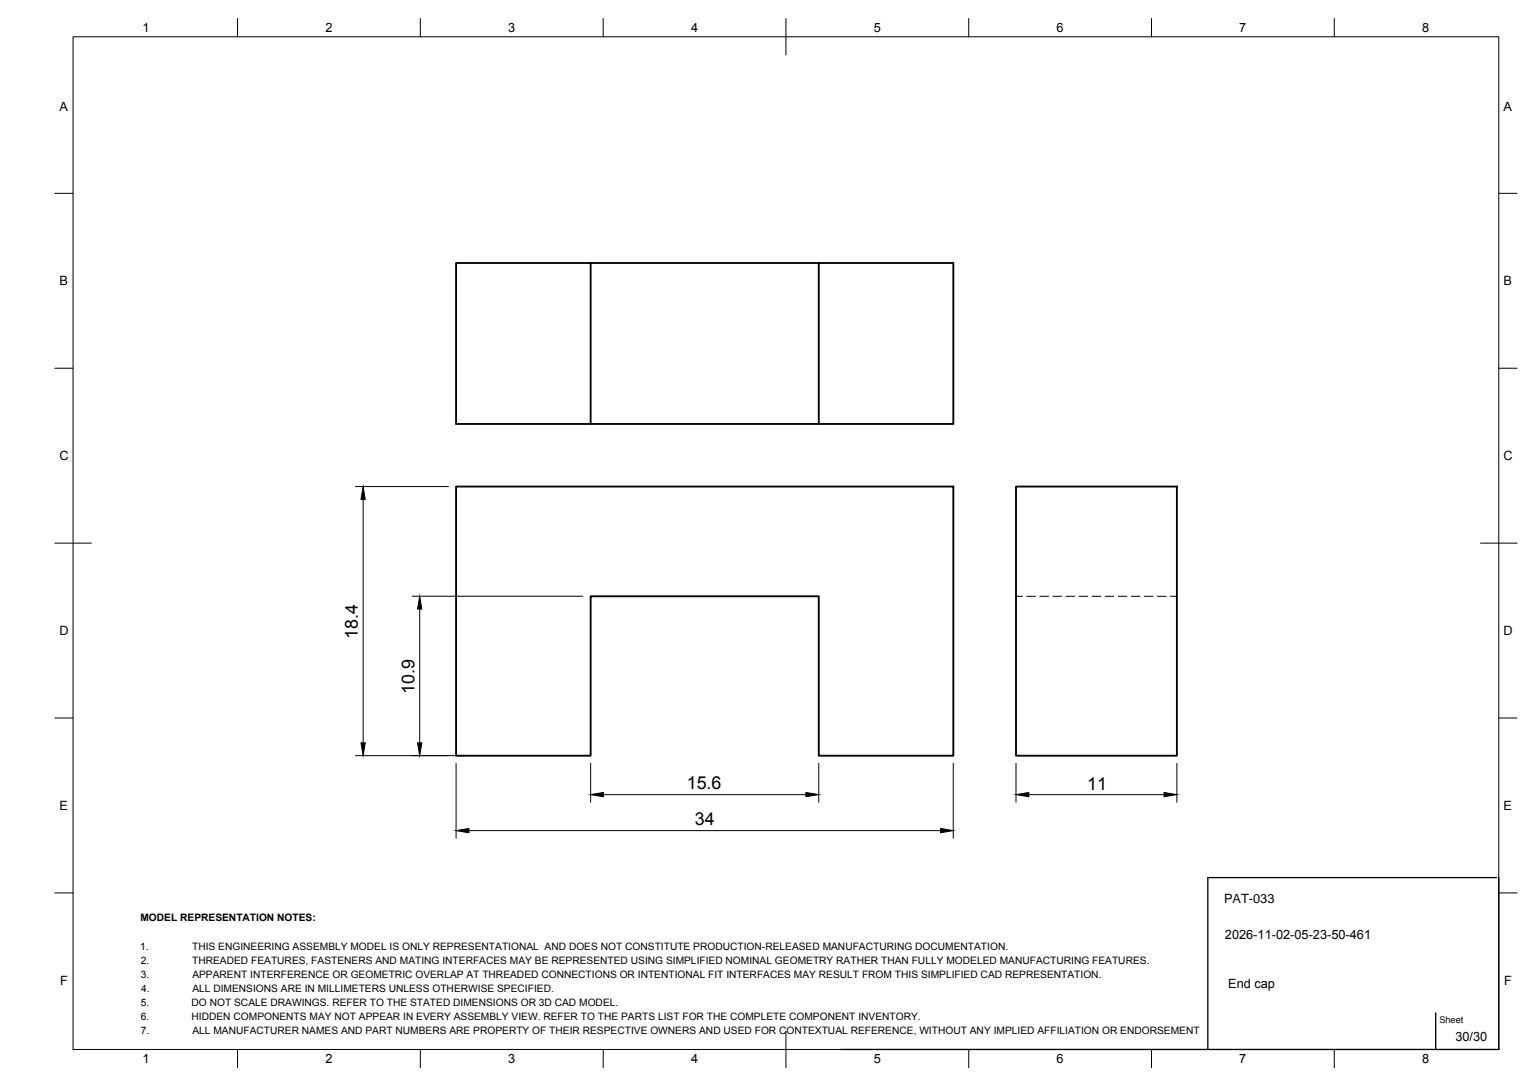
ISO-10303-21;
HEADER;
/* Generated by software containing ST-Developer
 * from STEP Tools, Inc. (www.steptools.com) 
 */

FILE_DESCRIPTION(
/* description */ ('Dual-rail gantry carriage'),
/* implementation_level */ '2;1');

FILE_NAME(
/* name */ 'End cap.step',
/* time_stamp */ '2026-10-27T10:49:15-07:00',
/* author */ (''),
/* organization */ (''),
/* preprocessor_version */ 'ST-DEVELOPER v20.2',
/* originating_system */ 'Autodesk Translation Framework v15.17.0.0',
/* authorisation */ '');

FILE_SCHEMA (('AUTOMOTIVE_DESIGN { 1 0 10303 214 3 1 1 }'));
ENDSEC;

DATA;
#10=MECHANICAL_DESIGN_GEOMETRIC_PRESENTATION_REPRESENTATION('',(#609),#12804);
#547=SHAPE_REPRESENTATION_RELATIONSHIP('SRR','None',#13027,#578);
#578=ADVANCED_BREP_SHAPE_REPRESENTATION('',(#638),#12797);
#609=STYLED_ITEM('',(#13261),#638);
#638=MANIFOLD_SOLID_BREP('Body1',#7389);
#999=PLANE('',#8250);
#1000=PLANE('',#8251);
#1001=PLANE('',#8252);
#1002=PLANE('',#8253);
#1003=PLANE('',#8254);
#1004=PLANE('',#8255);
#1005=PLANE('',#8256);
#1006=PLANE('',#8257);
#1007=PLANE('',#8258);
#1008=PLANE('',#8259);
#1363=FACE_OUTER_BOUND('',#1865,.T.);
#1364=FACE_OUTER_BOUND('',#1866,.T.);
#1365=FACE_OUTER_BOUND('',#1867,.T.);
#1366=FACE_OUTER_BOUND('',#1868,.T.);
#1367=FACE_OUTER_BOUND('',#1869,.T.);
#1368=FACE_OUTER_BOUND('',#1870,.T.);
#1369=FACE_OUTER_BOUND('',#1871,.T.);
#1370=FACE_OUTER_BOUND('',#1872,.T.);
#1371=FACE_OUTER_BOUND('',#1873,.T.);
#1372=FACE_OUTER_BOUND('',#1874,.T.);
#1865=EDGE_LOOP('',(#6609,#6610,#6611,#6612));
#1866=EDGE_LOOP('',(#6613,#6614,#6615,#6616));
#1867=EDGE_LOOP('',(#6617,#6618,#6619,#6620));
#1868=EDGE_LOOP('',(#6621,#6622,#6623,#6624));
#1869=EDGE_LOOP('',(#6625,#6626,#6627,#6628));
#1870=EDGE_LOOP('',(#6629,#6630,#6631,#6632));
#1871=EDGE_LOOP('',(#6633,#6634,#6635,#6636));
#1872=EDGE_LOOP('',(#6637,#6638,#6639,#6640));
#1873=EDGE_LOOP('',(#6641,#6642,#6643,#6644,#6645,#6646,#6647,#6648));
#1874=EDGE_LOOP('',(#6649,#6650,#6651,#6652,#6653,#6654,#6655,#6656));
#2554=LINE('',#12307,#3263);
#2555=LINE('',#12309,#3264);
#2556=LINE('',#12311,#3265);
#2557=LINE('',#12312,#3266);
#2558=LINE('',#12315,#3267);
#2559=LINE('',#12317,#3268);
#2560=LINE('',#12318,#3269);
#2561=LINE('',#12321,#3270);
#2562=LINE('',#12323,#3271);
#2563=LINE('',#12324,#3272);
#2564=LINE('',#12327,#3273);
#2565=LINE('',#12329,#3274);
#2566=LINE('',#12330,#3275);
#2567=LINE('',#12333,#3276);
#2568=LINE('',#12335,#3277);
#2569=LINE('',#12336,#3278);
#2570=LINE('',#12339,#3279);
#2571=LINE('',#12341,#3280);
#2572=LINE('',#12342,#3281);
#2573=LINE('',#12345,#3282);
#2574=LINE('',#12347,#3283);
#2575=LINE('',#12348,#3284);
#2576=LINE('',#12350,#3285);
#2577=LINE('',#12351,#3286);
#3263=VECTOR('',#10113,1.);
#3264=VECTOR('',#10114,1.);
#3265=VECTOR('',#10115,1.);
#3266=VECTOR('',#10116,1.);
#3267=VECTOR('',#10119,1.);
#3268=VECTOR('',#10120,1.);
#3269=VECTOR('',#10121,1.);
#3270=VECTOR('',#10124,1.);
#3271=VECTOR('',#10125,1.);
#3272=VECTOR('',#10126,1.);
#3273=VECTOR('',#10129,1.);
#3274=VECTOR('',#10130,1.);
#3275=VECTOR('',#10131,1.);
#3276=VECTOR('',#10134,1.);
#3277=VECTOR('',#10135,1.);
#3278=VECTOR('',#10136,1.);
#3279=VECTOR('',#10139,1.);
#3280=VECTOR('',#10140,1.);
#3281=VECTOR('',#10141,1.);
#3282=VECTOR('',#10144,1.);
#3283=VECTOR('',#10145,1.);
#3284=VECTOR('',#10146,1.);
#3285=VECTOR('',#10149,1.);
#3286=VECTOR('',#10150,1.);
#4067=VERTEX_POINT('',#12305);
#4068=VERTEX_POINT('',#12306);
#4069=VERTEX_POINT('',#12308);
#4070=VERTEX_POINT('',#12310);
#4071=VERTEX_POINT('',#12314);
#4072=VERTEX_POINT('',#12316);
#4073=VERTEX_POINT('',#12320);
#4074=VERTEX_POINT('',#12322);
#4075=VERTEX_POINT('',#12326);
#4076=VERTEX_POINT('',#12328);
#4077=VERTEX_POINT('',#12332);
#4078=VERTEX_POINT('',#12334);
#4079=VERTEX_POINT('',#12338);
#4080=VERTEX_POINT('',#12340);
#4081=VERTEX_POINT('',#12344);
#4082=VERTEX_POINT('',#12346);
#4927=EDGE_CURVE('',#4067,#4068,#2554,.T.);
#4928=EDGE_CURVE('',#4067,#4069,#2555,.T.);
#4929=EDGE_CURVE('',#4070,#4069,#2556,.T.);
#4930=EDGE_CURVE('',#4068,#4070,#2557,.T.);
#4931=EDGE_CURVE('',#4068,#4071,#2558,.T.);
#4932=EDGE_CURVE('',#4072,#4070,#2559,.T.);
#4933=EDGE_CURVE('',#4071,#4072,#2560,.T.);
#4934=EDGE_CURVE('',#4071,#4073,#2561,.T.);
#4935=EDGE_CURVE('',#4074,#4072,#2562,.T.);
#4936=EDGE_CURVE('',#4073,#4074,#2563,.T.);
#4937=EDGE_CURVE('',#4073,#4075,#2564,.T.);
#4938=EDGE_CURVE('',#4076,#4074,#2565,.T.);
#4939=EDGE_CURVE('',#4075,#4076,#2566,.T.);
#4940=EDGE_CURVE('',#4075,#4077,#2567,.T.);
#4941=EDGE_CURVE('',#4078,#4076,#2568,.T.);
#4942=EDGE_CURVE('',#4077,#4078,#2569,.T.);
#4943=EDGE_CURVE('',#4077,#4079,#2570,.T.);
#4944=EDGE_CURVE('',#4080,#4078,#2571,.T.);
#4945=EDGE_CURVE('',#4079,#4080,#2572,.T.);
#4946=EDGE_CURVE('',#4079,#4081,#2573,.T.);
#4947=EDGE_CURVE('',#4082,#4080,#2574,.T.);
#4948=EDGE_CURVE('',#4081,#4082,#2575,.T.);
#4949=EDGE_CURVE('',#4081,#4067,#2576,.T.);
#4950=EDGE_CURVE('',#4069,#4082,#2577,.T.);
#6609=ORIENTED_EDGE('',*,*,#4927,.F.);
#6610=ORIENTED_EDGE('',*,*,#4928,.T.);
#6611=ORIENTED_EDGE('',*,*,#4929,.F.);
#6612=ORIENTED_EDGE('',*,*,#4930,.F.);
#6613=ORIENTED_EDGE('',*,*,#4931,.F.);
#6614=ORIENTED_EDGE('',*,*,#4930,.T.);
#6615=ORIENTED_EDGE('',*,*,#4932,.F.);
#6616=ORIENTED_EDGE('',*,*,#4933,.F.);
#6617=ORIENTED_EDGE('',*,*,#4934,.F.);
#6618=ORIENTED_EDGE('',*,*,#4933,.T.);
#6619=ORIENTED_EDGE('',*,*,#4935,.F.);
#6620=ORIENTED_EDGE('',*,*,#4936,.F.);
#6621=ORIENTED_EDGE('',*,*,#4937,.F.);
#6622=ORIENTED_EDGE('',*,*,#4936,.T.);
#6623=ORIENTED_EDGE('',*,*,#4938,.F.);
#6624=ORIENTED_EDGE('',*,*,#4939,.F.);
#6625=ORIENTED_EDGE('',*,*,#4940,.F.);
#6626=ORIENTED_EDGE('',*,*,#4939,.T.);
#6627=ORIENTED_EDGE('',*,*,#4941,.F.);
#6628=ORIENTED_EDGE('',*,*,#4942,.F.);
#6629=ORIENTED_EDGE('',*,*,#4943,.F.);
#6630=ORIENTED_EDGE('',*,*,#4942,.T.);
#6631=ORIENTED_EDGE('',*,*,#4944,.F.);
#6632=ORIENTED_EDGE('',*,*,#4945,.F.);
#6633=ORIENTED_EDGE('',*,*,#4946,.F.);
#6634=ORIENTED_EDGE('',*,*,#4945,.T.);
#6635=ORIENTED_EDGE('',*,*,#4947,.F.);
#6636=ORIENTED_EDGE('',*,*,#4948,.F.);
#6637=ORIENTED_EDGE('',*,*,#4949,.F.);
#6638=ORIENTED_EDGE('',*,*,#4948,.T.);
#6639=ORIENTED_EDGE('',*,*,#4950,.F.);
#6640=ORIENTED_EDGE('',*,*,#4928,.F.);
#6641=ORIENTED_EDGE('',*,*,#4949,.T.);
#6642=ORIENTED_EDGE('',*,*,#4927,.T.);
#6643=ORIENTED_EDGE('',*,*,#4931,.T.);
#6644=ORIENTED_EDGE('',*,*,#4934,.T.);
#6645=ORIENTED_EDGE('',*,*,#4937,.T.);
#6646=ORIENTED_EDGE('',*,*,#4940,.T.);
#6647=ORIENTED_EDGE('',*,*,#4943,.T.);
#6648=ORIENTED_EDGE('',*,*,#4946,.T.);
#6649=ORIENTED_EDGE('',*,*,#4950,.T.);
#6650=ORIENTED_EDGE('',*,*,#4947,.T.);
#6651=ORIENTED_EDGE('',*,*,#4944,.T.);
#6652=ORIENTED_EDGE('',*,*,#4941,.T.);
#6653=ORIENTED_EDGE('',*,*,#4938,.T.);
#6654=ORIENTED_EDGE('',*,*,#4935,.T.);
#6655=ORIENTED_EDGE('',*,*,#4932,.T.);
#6656=ORIENTED_EDGE('',*,*,#4929,.T.);
#7289=ADVANCED_FACE('',(#1363),#999,.T.);
#7290=ADVANCED_FACE('',(#1364),#1000,.T.);
#7291=ADVANCED_FACE('',(#1365),#1001,.T.);
#7292=ADVANCED_FACE('',(#1366),#1002,.T.);
#7293=ADVANCED_FACE('',(#1367),#1003,.T.);
#7294=ADVANCED_FACE('',(#1368),#1004,.T.);
#7295=ADVANCED_FACE('',(#1369),#1005,.T.);
#7296=ADVANCED_FACE('',(#1370),#1006,.T.);
#7297=ADVANCED_FACE('',(#1371),#1007,.T.);
#7298=ADVANCED_FACE('',(#1372),#1008,.T.);
#7389=CLOSED_SHELL('',(#7289,#7290,#7291,#7292,#7293,#7294,#7295,#7296,
#7297,#7298));
#8249=AXIS2_PLACEMENT_3D('',#12303,#10109,#10110);
#8250=AXIS2_PLACEMENT_3D('',#12304,#10111,#10112);
#8251=AXIS2_PLACEMENT_3D('',#12313,#10117,#10118);
#8252=AXIS2_PLACEMENT_3D('',#12319,#10122,#10123);
#8253=AXIS2_PLACEMENT_3D('',#12325,#10127,#10128);
#8254=AXIS2_PLACEMENT_3D('',#12331,#10132,#10133);
#8255=AXIS2_PLACEMENT_3D('',#12337,#10137,#10138);
#8256=AXIS2_PLACEMENT_3D('',#12343,#10142,#10143);
#8257=AXIS2_PLACEMENT_3D('',#12349,#10147,#10148);
#8258=AXIS2_PLACEMENT_3D('',#12352,#10151,#10152);
#8259=AXIS2_PLACEMENT_3D('',#12353,#10153,#10154);
#10109=DIRECTION('axis',(0.,0.,1.));
#10110=DIRECTION('refdir',(1.,0.,0.));
#10111=DIRECTION('center_axis',(0.,0.,-1.));
#10112=DIRECTION('ref_axis',(0.,-1.,0.));
#10113=DIRECTION('',(0.,1.,0.));
#10114=DIRECTION('',(-1.,0.,0.));
#10115=DIRECTION('',(0.,-1.,0.));
#10116=DIRECTION('',(-1.,0.,0.));
#10117=DIRECTION('center_axis',(0.,1.,0.));
#10118=DIRECTION('ref_axis',(0.,0.,-1.));
#10119=DIRECTION('',(0.,0.,1.));
#10120=DIRECTION('',(0.,0.,-1.));
#10121=DIRECTION('',(-1.,0.,0.));
#10122=DIRECTION('center_axis',(0.,0.,-1.));
#10123=DIRECTION('ref_axis',(0.,-1.,0.));
#10124=DIRECTION('',(0.,1.,0.));
#10125=DIRECTION('',(0.,-1.,0.));
#10126=DIRECTION('',(-1.,0.,0.));
#10127=DIRECTION('center_axis',(0.,-1.,0.));
#10128=DIRECTION('ref_axis',(0.,0.,1.));
#10129=DIRECTION('',(0.,0.,-1.));
#10130=DIRECTION('',(0.,0.,1.));
#10131=DIRECTION('',(-1.,0.,0.));
#10132=DIRECTION('center_axis',(0.,0.,-1.));
#10133=DIRECTION('ref_axis',(0.,-1.,0.));
#10134=DIRECTION('',(0.,1.,0.));
#10135=DIRECTION('',(0.,-1.,0.));
#10136=DIRECTION('',(-1.,0.,0.));
#10137=DIRECTION('center_axis',(0.,1.,0.));
#10138=DIRECTION('ref_axis',(0.,0.,-1.));
#10139=DIRECTION('',(0.,0.,1.));
#10140=DIRECTION('',(0.,0.,-1.));
#10141=DIRECTION('',(-1.,0.,0.));
#10142=DIRECTION('center_axis',(0.,0.,1.));
#10143=DIRECTION('ref_axis',(0.,1.,0.));
#10144=DIRECTION('',(0.,-1.,0.));
#10145=DIRECTION('',(0.,1.,0.));
#10146=DIRECTION('',(-1.,0.,0.));
#10147=DIRECTION('center_axis',(0.,-1.,0.));
#10148=DIRECTION('ref_axis',(0.,0.,1.));
#10149=DIRECTION('',(0.,0.,-1.));
#10150=DIRECTION('',(0.,0.,1.));
#10151=DIRECTION('center_axis',(1.,0.,0.));
#10152=DIRECTION('ref_axis',(0.,0.,-1.));
#10153=DIRECTION('center_axis',(-1.,0.,0.));
#10154=DIRECTION('ref_axis',(0.,0.,1.));
#12303=CARTESIAN_POINT('',(0.,0.,0.));
#12304=CARTESIAN_POINT('Origin',(-1.97,-0.78,0.46));
#12305=CARTESIAN_POINT('',(-1.97,-1.7,0.46));
#12306=CARTESIAN_POINT('',(-1.97,-0.78,0.46));
#12307=CARTESIAN_POINT('',(-1.97,-1.7,0.46));
#12308=CARTESIAN_POINT('',(-3.07,-1.7,0.46));
#12309=CARTESIAN_POINT('',(-1.97,-1.7,0.46));
#12310=CARTESIAN_POINT('',(-3.07,-0.78,0.46));
#12311=CARTESIAN_POINT('',(-3.07,-1.7,0.46));
#12312=CARTESIAN_POINT('',(-1.97,-0.78,0.46));
#12313=CARTESIAN_POINT('Origin',(-1.97,-0.78,1.55));
#12314=CARTESIAN_POINT('',(-1.97,-0.78,1.55));
#12315=CARTESIAN_POINT('',(-1.97,-0.78,0.46));
#12316=CARTESIAN_POINT('',(-3.07,-0.78,1.55));
#12317=CARTESIAN_POINT('',(-3.07,-0.78,0.46));
#12318=CARTESIAN_POINT('',(-1.97,-0.78,1.55));
#12319=CARTESIAN_POINT('Origin',(-1.97,0.78,1.55));
#12320=CARTESIAN_POINT('',(-1.97,0.78,1.55));
#12321=CARTESIAN_POINT('',(-1.97,-0.78,1.55));
#12322=CARTESIAN_POINT('',(-3.07,0.78,1.55));
#12323=CARTESIAN_POINT('',(-3.07,-0.78,1.55));
#12324=CARTESIAN_POINT('',(-1.97,0.78,1.55));
#12325=CARTESIAN_POINT('Origin',(-1.97,0.78,0.46));
#12326=CARTESIAN_POINT('',(-1.97,0.78,0.46));
#12327=CARTESIAN_POINT('',(-1.97,0.78,1.55));
#12328=CARTESIAN_POINT('',(-3.07,0.78,0.46));
#12329=CARTESIAN_POINT('',(-3.07,0.78,1.55));
#12330=CARTESIAN_POINT('',(-1.97,0.78,0.46));
#12331=CARTESIAN_POINT('Origin',(-1.97,1.7,0.46));
#12332=CARTESIAN_POINT('',(-1.97,1.7,0.46));
#12333=CARTESIAN_POINT('',(-1.97,0.78,0.46));
#12334=CARTESIAN_POINT('',(-3.07,1.7,0.46));
#12335=CARTESIAN_POINT('',(-3.07,0.78,0.46));
#12336=CARTESIAN_POINT('',(-1.97,1.7,0.46));
#12337=CARTESIAN_POINT('Origin',(-1.97,1.7,2.3));
#12338=CARTESIAN_POINT('',(-1.97,1.7,2.3));
#12339=CARTESIAN_POINT('',(-1.97,1.7,0.46));
#12340=CARTESIAN_POINT('',(-3.07,1.7,2.3));
#12341=CARTESIAN_POINT('',(-3.07,1.7,0.46));
#12342=CARTESIAN_POINT('',(-1.97,1.7,2.3));
#12343=CARTESIAN_POINT('Origin',(-1.97,-1.7,2.3));
#12344=CARTESIAN_POINT('',(-1.97,-1.7,2.3));
#12345=CARTESIAN_POINT('',(-1.97,1.7,2.3));
#12346=CARTESIAN_POINT('',(-3.07,-1.7,2.3));
#12347=CARTESIAN_POINT('',(-3.07,1.7,2.3));
#12348=CARTESIAN_POINT('',(-1.97,-1.7,2.3));
#12349=CARTESIAN_POINT('Origin',(-1.97,-1.7,0.46));
#12350=CARTESIAN_POINT('',(-1.97,-1.7,2.3));
#12351=CARTESIAN_POINT('',(-3.07,-1.7,2.3));
#12352=CARTESIAN_POINT('Origin',(-1.97,0.,1.38));
#12353=CARTESIAN_POINT('Origin',(-3.07,0.,1.38));
#12761=UNCERTAINTY_MEASURE_WITH_UNIT(LENGTH_MEASURE(0.001),#12805,
'DISTANCE_ACCURACY_VALUE',
'Maximum model space distance between geometric entities at asserted c
onnectivities');
#12768=UNCERTAINTY_MEASURE_WITH_UNIT(LENGTH_MEASURE(0.001),#12805,
'DISTANCE_ACCURACY_VALUE',
'Maximum model space distance between geometric entities at asserted c
onnectivities');
#12797=(
GEOMETRIC_REPRESENTATION_CONTEXT(3)
GLOBAL_UNCERTAINTY_ASSIGNED_CONTEXT((#12761))
GLOBAL_UNIT_ASSIGNED_CONTEXT((#12805,#12807,#12808))
REPRESENTATION_CONTEXT('','3D')
);
#12804=(
GEOMETRIC_REPRESENTATION_CONTEXT(3)
GLOBAL_UNCERTAINTY_ASSIGNED_CONTEXT((#12768))
GLOBAL_UNIT_ASSIGNED_CONTEXT((#12805,#12807,#12808))
REPRESENTATION_CONTEXT('','3D')
);
#12805=(
LENGTH_UNIT()
NAMED_UNIT(*)
SI_UNIT(.CENTI.,.METRE.)
);
#12807=(
NAMED_UNIT(*)
PLANE_ANGLE_UNIT()
SI_UNIT($,.RADIAN.)
);
#12808=(
NAMED_UNIT(*)
SI_UNIT($,.STERADIAN.)
SOLID_ANGLE_UNIT()
);
#12837=SHAPE_DEFINITION_REPRESENTATION(#12872,#13027);
#12872=PRODUCT_DEFINITION_SHAPE('',$,#13063);
#13027=SHAPE_REPRESENTATION('',(#8249),#12797);
#13034=PRODUCT_DEFINITION_CONTEXT('part definition',#13141,'design');
#13063=PRODUCT_DEFINITION('End cap','End cap',#13098,#13034);
#13098=PRODUCT_DEFINITION_FORMATION('',$,#13171);
#13141=APPLICATION_CONTEXT(
'Core Data for Automotive Mechanical Design Process');
#13142=PRODUCT_CONTEXT('part definition',#13141,'mechanical');
#13171=PRODUCT('End cap','End cap','End cap',(#13142));
#13255=COLOUR_RGB('Off White',0.89,0.88,0.83);
#13256=FILL_AREA_STYLE_COLOUR('',#13255);
#13257=FILL_AREA_STYLE('',(#13256));
#13258=SURFACE_STYLE_FILL_AREA(#13257);
#13259=SURFACE_SIDE_STYLE('',(#13258));
#13260=SURFACE_STYLE_USAGE(.BOTH.,#13259);
#13261=PRESENTATION_STYLE_ASSIGNMENT((#13260));
ENDSEC;
END-ISO-10303-21;
